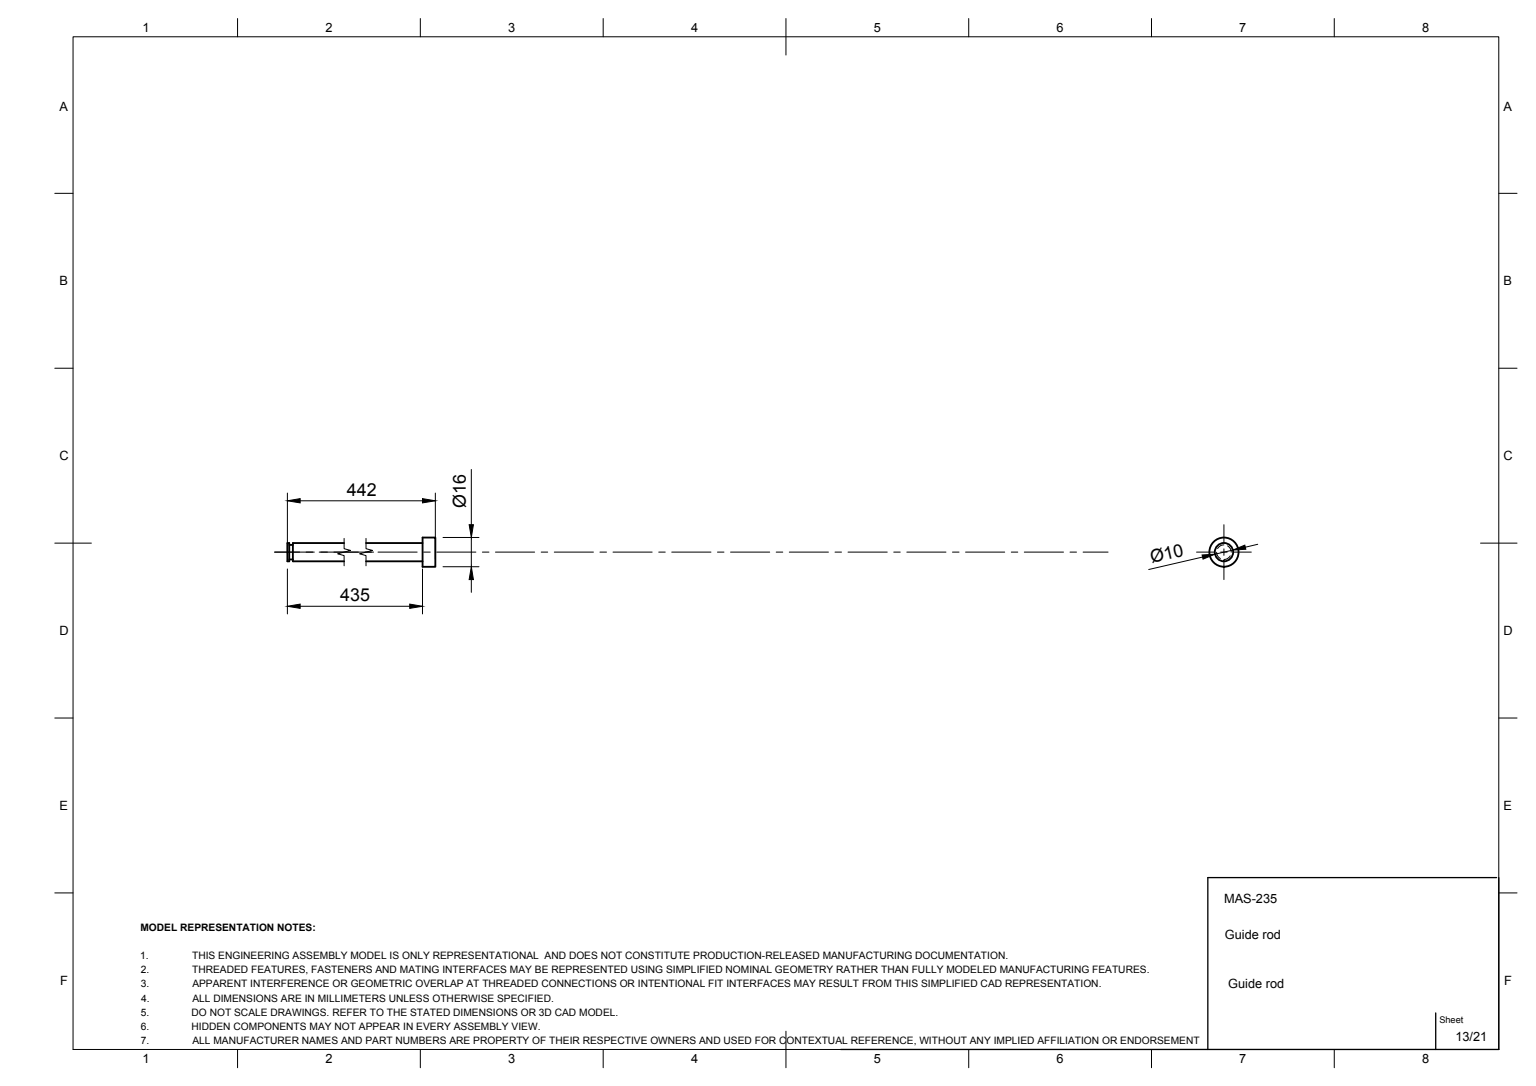
ISO-10303-21;
HEADER;
/* Generated by software containing ST-Developer
 * from STEP Tools, Inc. (www.steptools.com) 
 */

FILE_DESCRIPTION(
/* description */ ('Independent Whitworth quick-return mechanism. Crank radius40, ground-
center spacing80, lever180, connecting rod160, output guide X200. Nomi
nal stroke180 and long/short phase ratio2. Retained guide rods, replac
eable bearing sleeves and captured sliding shoe. No load or production
 rating assigned.'),
/* implementation_level */ '2;1');

FILE_NAME(
/* name */ 'Guide rod.step',
/* time_stamp */ '2026-11-09T18:22:56-08:00',
/* author */ (''),
/* organization */ (''),
/* preprocessor_version */ 'ST-DEVELOPER v20.2',
/* originating_system */ 'Autodesk Translation Framework v15.17.0.0',
/* authorisation */ '');

FILE_SCHEMA (('AUTOMOTIVE_DESIGN { 1 0 10303 214 3 1 1 }'));
ENDSEC;

DATA;
#10=MECHANICAL_DESIGN_GEOMETRIC_PRESENTATION_REPRESENTATION('',(#229),#4388);
#189=SHAPE_REPRESENTATION_RELATIONSHIP('SRR','None',#4488,#209);
#209=ADVANCED_BREP_SHAPE_REPRESENTATION('',(#249),#4378);
#229=STYLED_ITEM('',(#4595),#249);
#249=MANIFOLD_SOLID_BREP('Body1',#2334);
#293=FACE_BOUND('',#659,.T.);
#294=FACE_BOUND('',#661,.T.);
#295=FACE_BOUND('',#664,.T.);
#363=PLANE('',#2705);
#364=PLANE('',#2707);
#365=PLANE('',#2711);
#366=PLANE('',#2716);
#367=PLANE('',#2718);
#476=FACE_OUTER_BOUND('',#657,.T.);
#477=FACE_OUTER_BOUND('',#658,.T.);
#478=FACE_OUTER_BOUND('',#660,.T.);
#479=FACE_OUTER_BOUND('',#662,.T.);
#480=FACE_OUTER_BOUND('',#663,.T.);
#481=FACE_OUTER_BOUND('',#665,.T.);
#482=FACE_OUTER_BOUND('',#666,.T.);
#483=FACE_OUTER_BOUND('',#667,.T.);
#484=FACE_OUTER_BOUND('',#668,.T.);
#657=EDGE_LOOP('',(#1900,#1901,#1902,#1903));
#658=EDGE_LOOP('',(#1904));
#659=EDGE_LOOP('',(#1905));
#660=EDGE_LOOP('',(#1906));
#661=EDGE_LOOP('',(#1907));
#662=EDGE_LOOP('',(#1908,#1909,#1910,#1911));
#663=EDGE_LOOP('',(#1912));
#664=EDGE_LOOP('',(#1913));
#665=EDGE_LOOP('',(#1914,#1915,#1916,#1917));
#666=EDGE_LOOP('',(#1918));
#667=EDGE_LOOP('',(#1919,#1920,#1921,#1922));
#668=EDGE_LOOP('',(#1923));
#858=LINE('',#4042,#997);
#859=LINE('',#4053,#998);
#860=LINE('',#4061,#999);
#861=LINE('',#4065,#1000);
#997=VECTOR('',#3274,4.);
#998=VECTOR('',#3289,5.);
#999=VECTOR('',#3298,8.);
#1000=VECTOR('',#3305,5.);
#1091=CIRCLE('',#2703,4.);
#1092=CIRCLE('',#2704,4.);
#1093=CIRCLE('',#2706,5.);
#1094=CIRCLE('',#2708,5.);
#1095=CIRCLE('',#2710,5.);
#1096=CIRCLE('',#2712,8.);
#1097=CIRCLE('',#2713,5.);
#1098=CIRCLE('',#2715,8.);
#1261=VERTEX_POINT('',#4039);
#1262=VERTEX_POINT('',#4041);
#1263=VERTEX_POINT('',#4045);
#1264=VERTEX_POINT('',#4048);
#1265=VERTEX_POINT('',#4051);
#1266=VERTEX_POINT('',#4055);
#1267=VERTEX_POINT('',#4057);
#1268=VERTEX_POINT('',#4060);
#1486=EDGE_CURVE('',#1261,#1261,#1091,.T.);
#1487=EDGE_CURVE('',#1261,#1262,#858,.T.);
#1488=EDGE_CURVE('',#1262,#1262,#1092,.T.);
#1489=EDGE_CURVE('',#1263,#1263,#1093,.T.);
#1490=EDGE_CURVE('',#1264,#1264,#1094,.T.);
#1491=EDGE_CURVE('',#1265,#1265,#1095,.T.);
#1492=EDGE_CURVE('',#1265,#1264,#859,.T.);
#1493=EDGE_CURVE('',#1266,#1266,#1096,.T.);
#1494=EDGE_CURVE('',#1267,#1267,#1097,.T.);
#1495=EDGE_CURVE('',#1266,#1268,#860,.T.);
#1496=EDGE_CURVE('',#1268,#1268,#1098,.T.);
#1497=EDGE_CURVE('',#1263,#1267,#861,.T.);
#1900=ORIENTED_EDGE('',*,*,#1486,.T.);
#1901=ORIENTED_EDGE('',*,*,#1487,.T.);
#1902=ORIENTED_EDGE('',*,*,#1488,.F.);
#1903=ORIENTED_EDGE('',*,*,#1487,.F.);
#1904=ORIENTED_EDGE('',*,*,#1489,.F.);
#1905=ORIENTED_EDGE('',*,*,#1486,.F.);
#1906=ORIENTED_EDGE('',*,*,#1490,.F.);
#1907=ORIENTED_EDGE('',*,*,#1488,.T.);
#1908=ORIENTED_EDGE('',*,*,#1491,.F.);
#1909=ORIENTED_EDGE('',*,*,#1492,.T.);
#1910=ORIENTED_EDGE('',*,*,#1490,.T.);
#1911=ORIENTED_EDGE('',*,*,#1492,.F.);
#1912=ORIENTED_EDGE('',*,*,#1493,.T.);
#1913=ORIENTED_EDGE('',*,*,#1494,.F.);
#1914=ORIENTED_EDGE('',*,*,#1493,.F.);
#1915=ORIENTED_EDGE('',*,*,#1495,.T.);
#1916=ORIENTED_EDGE('',*,*,#1496,.T.);
#1917=ORIENTED_EDGE('',*,*,#1495,.F.);
#1918=ORIENTED_EDGE('',*,*,#1496,.F.);
#1919=ORIENTED_EDGE('',*,*,#1489,.T.);
#1920=ORIENTED_EDGE('',*,*,#1497,.T.);
#1921=ORIENTED_EDGE('',*,*,#1494,.T.);
#1922=ORIENTED_EDGE('',*,*,#1497,.F.);
#1923=ORIENTED_EDGE('',*,*,#1491,.T.);
#2143=CYLINDRICAL_SURFACE('',#2702,4.);
#2144=CYLINDRICAL_SURFACE('',#2709,5.);
#2145=CYLINDRICAL_SURFACE('',#2714,8.);
#2146=CYLINDRICAL_SURFACE('',#2717,5.);
#2248=ADVANCED_FACE('',(#476),#2143,.T.);
#2249=ADVANCED_FACE('',(#477,#293),#363,.F.);
#2250=ADVANCED_FACE('',(#478,#294),#364,.F.);
#2251=ADVANCED_FACE('',(#479),#2144,.T.);
#2252=ADVANCED_FACE('',(#480,#295),#365,.T.);
#2253=ADVANCED_FACE('',(#481),#2145,.T.);
#2254=ADVANCED_FACE('',(#482),#366,.F.);
#2255=ADVANCED_FACE('',(#483),#2146,.T.);
#2256=ADVANCED_FACE('',(#484),#367,.T.);
#2334=CLOSED_SHELL('',(#2248,#2249,#2250,#2251,#2252,#2253,#2254,#2255,
#2256));
#2701=AXIS2_PLACEMENT_3D('',#4037,#3268,#3269);
#2702=AXIS2_PLACEMENT_3D('',#4038,#3270,#3271);
#2703=AXIS2_PLACEMENT_3D('',#4040,#3272,#3273);
#2704=AXIS2_PLACEMENT_3D('',#4043,#3275,#3276);
#2705=AXIS2_PLACEMENT_3D('',#4044,#3277,#3278);
#2706=AXIS2_PLACEMENT_3D('',#4046,#3279,#3280);
#2707=AXIS2_PLACEMENT_3D('',#4047,#3281,#3282);
#2708=AXIS2_PLACEMENT_3D('',#4049,#3283,#3284);
#2709=AXIS2_PLACEMENT_3D('',#4050,#3285,#3286);
#2710=AXIS2_PLACEMENT_3D('',#4052,#3287,#3288);
#2711=AXIS2_PLACEMENT_3D('',#4054,#3290,#3291);
#2712=AXIS2_PLACEMENT_3D('',#4056,#3292,#3293);
#2713=AXIS2_PLACEMENT_3D('',#4058,#3294,#3295);
#2714=AXIS2_PLACEMENT_3D('',#4059,#3296,#3297);
#2715=AXIS2_PLACEMENT_3D('',#4062,#3299,#3300);
#2716=AXIS2_PLACEMENT_3D('',#4063,#3301,#3302);
#2717=AXIS2_PLACEMENT_3D('',#4064,#3303,#3304);
#2718=AXIS2_PLACEMENT_3D('',#4066,#3306,#3307);
#3268=DIRECTION('axis',(0.,0.,1.));
#3269=DIRECTION('refdir',(1.,0.,0.));
#3270=DIRECTION('center_axis',(0.,0.,1.));
#3271=DIRECTION('ref_axis',(1.,0.,0.));
#3272=DIRECTION('center_axis',(0.,0.,1.));
#3273=DIRECTION('ref_axis',(1.,0.,0.));
#3274=DIRECTION('',(0.,0.,1.));
#3275=DIRECTION('center_axis',(0.,0.,1.));
#3276=DIRECTION('ref_axis',(1.,0.,0.));
#3277=DIRECTION('center_axis',(0.,0.,-1.));
#3278=DIRECTION('ref_axis',(-1.,0.,0.));
#3279=DIRECTION('center_axis',(0.,0.,-1.));
#3280=DIRECTION('ref_axis',(1.,0.,0.));
#3281=DIRECTION('center_axis',(0.,0.,1.));
#3282=DIRECTION('ref_axis',(1.,0.,0.));
#3283=DIRECTION('center_axis',(0.,0.,1.));
#3284=DIRECTION('ref_axis',(1.,0.,0.));
#3285=DIRECTION('center_axis',(0.,0.,1.));
#3286=DIRECTION('ref_axis',(1.,0.,0.));
#3287=DIRECTION('center_axis',(0.,0.,1.));
#3288=DIRECTION('ref_axis',(1.,0.,0.));
#3289=DIRECTION('',(0.,0.,-1.));
#3290=DIRECTION('center_axis',(0.,0.,1.));
#3291=DIRECTION('ref_axis',(1.,0.,0.));
#3292=DIRECTION('center_axis',(0.,0.,1.));
#3293=DIRECTION('ref_axis',(1.,0.,0.));
#3294=DIRECTION('center_axis',(0.,0.,1.));
#3295=DIRECTION('ref_axis',(1.,0.,0.));
#3296=DIRECTION('center_axis',(0.,0.,1.));
#3297=DIRECTION('ref_axis',(1.,0.,0.));
#3298=DIRECTION('',(0.,0.,-1.));
#3299=DIRECTION('center_axis',(0.,0.,1.));
#3300=DIRECTION('ref_axis',(1.,0.,0.));
#3301=DIRECTION('center_axis',(0.,0.,1.));
#3302=DIRECTION('ref_axis',(1.,0.,0.));
#3303=DIRECTION('center_axis',(0.,0.,1.));
#3304=DIRECTION('ref_axis',(1.,0.,0.));
#3305=DIRECTION('',(0.,0.,-1.));
#3306=DIRECTION('center_axis',(0.,0.,1.));
#3307=DIRECTION('ref_axis',(1.,0.,0.));
#4037=CARTESIAN_POINT('',(0.,0.,0.));
#4038=CARTESIAN_POINT('Origin',(0.,0.,433.));
#4039=CARTESIAN_POINT('',(-4.,-4.89858719658941E-16,432.));
#4040=CARTESIAN_POINT('Origin',(0.,0.,432.));
#4041=CARTESIAN_POINT('',(-4.,-4.89858719658941E-16,434.));
#4042=CARTESIAN_POINT('',(-4.,-4.89858719658941E-16,433.));
#4043=CARTESIAN_POINT('Origin',(0.,0.,434.));
#4044=CARTESIAN_POINT('Origin',(8.,0.,432.));
#4045=CARTESIAN_POINT('',(-5.,6.12323399573677E-16,432.));
#4046=CARTESIAN_POINT('Origin',(0.,0.,432.));
#4047=CARTESIAN_POINT('Origin',(4.,0.,434.));
#4048=CARTESIAN_POINT('',(-5.,-6.12323399573677E-16,434.));
#4049=CARTESIAN_POINT('Origin',(0.,0.,434.));
#4050=CARTESIAN_POINT('Origin',(0.,0.,0.));
#4051=CARTESIAN_POINT('',(-5.,-6.12323399573677E-16,435.));
#4052=CARTESIAN_POINT('Origin',(0.,0.,435.));
#4053=CARTESIAN_POINT('',(-5.,-6.12323399573677E-16,0.));
#4054=CARTESIAN_POINT('Origin',(0.,0.,0.));
#4055=CARTESIAN_POINT('',(-8.,-9.79717439317883E-16,0.));
#4056=CARTESIAN_POINT('Origin',(0.,0.,0.));
#4057=CARTESIAN_POINT('',(-5.,-6.12323399573677E-16,0.));
#4058=CARTESIAN_POINT('Origin',(0.,0.,0.));
#4059=CARTESIAN_POINT('Origin',(0.,0.,-2.));
#4060=CARTESIAN_POINT('',(-8.,-9.79717439317883E-16,-7.));
#4061=CARTESIAN_POINT('',(-8.,-9.79717439317883E-16,-2.));
#4062=CARTESIAN_POINT('Origin',(0.,0.,-7.));
#4063=CARTESIAN_POINT('Origin',(0.,0.,-7.));
#4064=CARTESIAN_POINT('Origin',(0.,0.,0.));
#4065=CARTESIAN_POINT('',(-5.,-6.12323399573677E-16,0.));
#4066=CARTESIAN_POINT('Origin',(0.,0.,435.));
#4356=UNCERTAINTY_MEASURE_WITH_UNIT(LENGTH_MEASURE(0.01),#4389,
'DISTANCE_ACCURACY_VALUE',
'Maximum model space distance between geometric entities at asserted c
onnectivities');
#4366=UNCERTAINTY_MEASURE_WITH_UNIT(LENGTH_MEASURE(0.01),#4389,
'DISTANCE_ACCURACY_VALUE',
'Maximum model space distance between geometric entities at asserted c
onnectivities');
#4378=(
GEOMETRIC_REPRESENTATION_CONTEXT(3)
GLOBAL_UNCERTAINTY_ASSIGNED_CONTEXT((#4356))
GLOBAL_UNIT_ASSIGNED_CONTEXT((#4389,#4391,#4392))
REPRESENTATION_CONTEXT('','3D')
);
#4388=(
GEOMETRIC_REPRESENTATION_CONTEXT(3)
GLOBAL_UNCERTAINTY_ASSIGNED_CONTEXT((#4366))
GLOBAL_UNIT_ASSIGNED_CONTEXT((#4389,#4391,#4392))
REPRESENTATION_CONTEXT('','3D')
);
#4389=(
LENGTH_UNIT()
NAMED_UNIT(*)
SI_UNIT(.MILLI.,.METRE.)
);
#4391=(
NAMED_UNIT(*)
PLANE_ANGLE_UNIT()
SI_UNIT($,.RADIAN.)
);
#4392=(
NAMED_UNIT(*)
SI_UNIT($,.STERADIAN.)
SOLID_ANGLE_UNIT()
);
#4404=SHAPE_DEFINITION_REPRESENTATION(#4425,#4488);
#4425=PRODUCT_DEFINITION_SHAPE('',$,#4510);
#4488=SHAPE_REPRESENTATION('',(#2701),#4378);
#4498=PRODUCT_DEFINITION_CONTEXT('part definition',#4563,'design');
#4510=PRODUCT_DEFINITION('Guide rod','Guide rod',#4531,#4498);
#4531=PRODUCT_DEFINITION_FORMATION('',$,#4576);
#4563=APPLICATION_CONTEXT(
'Core Data for Automotive Mechanical Design Process');
#4564=PRODUCT_CONTEXT('part definition',#4563,'mechanical');
#4576=PRODUCT('Guide rod','Guide rod',$,(#4564));
#4595=PRESENTATION_STYLE_ASSIGNMENT((#4609));
#4609=SURFACE_STYLE_USAGE(.BOTH.,#4623);
#4623=SURFACE_SIDE_STYLE('',(#4637));
#4637=SURFACE_STYLE_FILL_AREA(#4651);
#4651=FILL_AREA_STYLE('Pivot gray',(#4665));
#4665=FILL_AREA_STYLE_COLOUR('Pivot gray',#4679);
#4679=COLOUR_RGB('Pivot gray',0.407843137254902,0.447058823529412,0.498039215686275);
ENDSEC;
END-ISO-10303-21;
